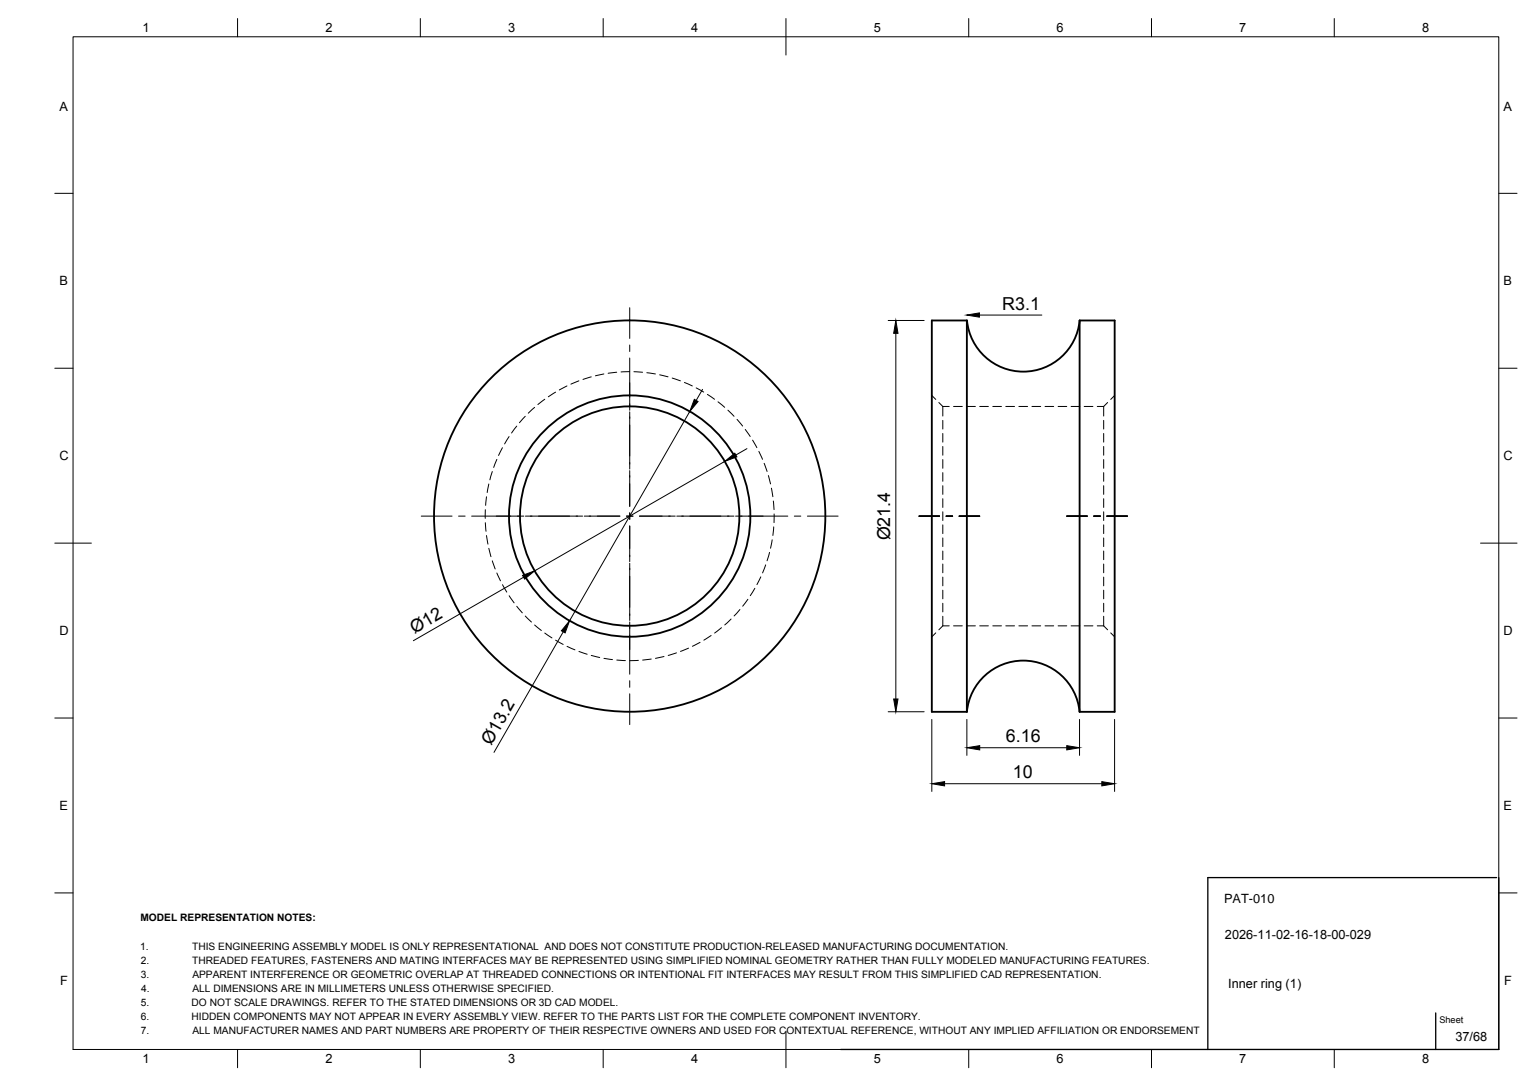
ISO-10303-21;
HEADER;
/* Generated by software containing ST-Developer
 * from STEP Tools, Inc. (www.steptools.com) 
 */

FILE_DESCRIPTION(
/* description */ ('Belt conveyor head drive unit'),
/* implementation_level */ '2;1');

FILE_NAME(
/* name */ 'Inner ring (1).step',
/* time_stamp */ '2026-10-28T03:26:19-07:00',
/* author */ (''),
/* organization */ (''),
/* preprocessor_version */ 'ST-DEVELOPER v20.2',
/* originating_system */ 'Autodesk Translation Framework v15.17.0.0',
/* authorisation */ '');

FILE_SCHEMA (('AUTOMOTIVE_DESIGN { 1 0 10303 214 3 1 1 }'));
ENDSEC;

DATA;
#10=MECHANICAL_DESIGN_GEOMETRIC_PRESENTATION_REPRESENTATION('',(#888),#27069);
#685=CONICAL_SURFACE('',#15366,0.63,0.785398163397448);
#686=CONICAL_SURFACE('',#15373,0.63,0.785398163397448);
#707=TOROIDAL_SURFACE('',#15355,1.1,0.309556);
#742=SHAPE_REPRESENTATION_RELATIONSHIP('SRR','None',#27388,#811);
#811=ADVANCED_BREP_SHAPE_REPRESENTATION('',(#972),#27030);
#888=STYLED_ITEM('',(#27797),#972);
#972=MANIFOLD_SOLID_BREP('Body1',#13754);
#1162=FACE_BOUND('',#2960,.T.);
#1163=FACE_BOUND('',#2963,.T.);
#1466=PLANE('',#15368);
#1467=PLANE('',#15371);
#2005=FACE_OUTER_BOUND('',#2955,.T.);
#2006=FACE_OUTER_BOUND('',#2956,.T.);
#2007=FACE_OUTER_BOUND('',#2957,.T.);
#2008=FACE_OUTER_BOUND('',#2958,.T.);
#2009=FACE_OUTER_BOUND('',#2959,.T.);
#2010=FACE_OUTER_BOUND('',#2961,.T.);
#2011=FACE_OUTER_BOUND('',#2962,.T.);
#2012=FACE_OUTER_BOUND('',#2964,.T.);
#2955=EDGE_LOOP('',(#10554,#10555,#10556,#10557,#10558,#10559));
#2956=EDGE_LOOP('',(#10560,#10561,#10562,#10563,#10564));
#2957=EDGE_LOOP('',(#10565,#10566,#10567,#10568));
#2958=EDGE_LOOP('',(#10569,#10570,#10571,#10572));
#2959=EDGE_LOOP('',(#10573));
#2960=EDGE_LOOP('',(#10574));
#2961=EDGE_LOOP('',(#10575,#10576,#10577,#10578,#10579));
#2962=EDGE_LOOP('',(#10580));
#2963=EDGE_LOOP('',(#10581));
#2964=EDGE_LOOP('',(#10582,#10583,#10584,#10585));
#3900=LINE('',#23073,#4692);
#3901=LINE('',#23079,#4693);
#3902=LINE('',#23083,#4694);
#3903=LINE('',#23089,#4695);
#3904=LINE('',#23094,#4696);
#4692=VECTOR('',#18436,1.070235);
#4693=VECTOR('',#18443,0.6);
#4694=VECTOR('',#18448,0.63);
#4695=VECTOR('',#18457,1.070235);
#4696=VECTOR('',#18464,0.63);
#5460=CIRCLE('',#15356,1.070235);
#5461=CIRCLE('',#15357,1.070235);
#5462=CIRCLE('',#15358,0.309556);
#5463=CIRCLE('',#15359,1.070235);
#5464=CIRCLE('',#15360,1.070235);
#5465=CIRCLE('',#15362,1.070235);
#5466=CIRCLE('',#15364,0.6);
#5467=CIRCLE('',#15365,0.6);
#5468=CIRCLE('',#15367,0.66);
#5469=CIRCLE('',#15370,1.070235);
#5470=CIRCLE('',#15372,0.66);
#6493=VERTEX_POINT('',#23062);
#6494=VERTEX_POINT('',#23063);
#6495=VERTEX_POINT('',#23066);
#6496=VERTEX_POINT('',#23068);
#6497=VERTEX_POINT('',#23072);
#6498=VERTEX_POINT('',#23076);
#6499=VERTEX_POINT('',#23078);
#6500=VERTEX_POINT('',#23082);
#6501=VERTEX_POINT('',#23087);
#6502=VERTEX_POINT('',#23091);
#7969=EDGE_CURVE('',#6493,#6494,#5460,.T.);
#7970=EDGE_CURVE('',#6494,#6493,#5461,.T.);
#7971=EDGE_CURVE('',#6494,#6495,#5462,.T.);
#7972=EDGE_CURVE('',#6496,#6495,#5463,.T.);
#7973=EDGE_CURVE('',#6495,#6496,#5464,.T.);
#7974=EDGE_CURVE('',#6496,#6497,#3900,.T.);
#7975=EDGE_CURVE('',#6497,#6497,#5465,.T.);
#7976=EDGE_CURVE('',#6498,#6498,#5466,.T.);
#7977=EDGE_CURVE('',#6498,#6499,#3901,.T.);
#7978=EDGE_CURVE('',#6499,#6499,#5467,.T.);
#7979=EDGE_CURVE('',#6499,#6500,#3902,.T.);
#7980=EDGE_CURVE('',#6500,#6500,#5468,.T.);
#7981=EDGE_CURVE('',#6501,#6501,#5469,.T.);
#7982=EDGE_CURVE('',#6501,#6493,#3903,.T.);
#7983=EDGE_CURVE('',#6502,#6502,#5470,.T.);
#7984=EDGE_CURVE('',#6502,#6498,#3904,.T.);
#10554=ORIENTED_EDGE('',*,*,#7969,.F.);
#10555=ORIENTED_EDGE('',*,*,#7970,.F.);
#10556=ORIENTED_EDGE('',*,*,#7971,.T.);
#10557=ORIENTED_EDGE('',*,*,#7972,.F.);
#10558=ORIENTED_EDGE('',*,*,#7973,.F.);
#10559=ORIENTED_EDGE('',*,*,#7971,.F.);
#10560=ORIENTED_EDGE('',*,*,#7972,.T.);
#10561=ORIENTED_EDGE('',*,*,#7973,.T.);
#10562=ORIENTED_EDGE('',*,*,#7974,.T.);
#10563=ORIENTED_EDGE('',*,*,#7975,.T.);
#10564=ORIENTED_EDGE('',*,*,#7974,.F.);
#10565=ORIENTED_EDGE('',*,*,#7976,.T.);
#10566=ORIENTED_EDGE('',*,*,#7977,.T.);
#10567=ORIENTED_EDGE('',*,*,#7978,.F.);
#10568=ORIENTED_EDGE('',*,*,#7977,.F.);
#10569=ORIENTED_EDGE('',*,*,#7978,.T.);
#10570=ORIENTED_EDGE('',*,*,#7979,.T.);
#10571=ORIENTED_EDGE('',*,*,#7980,.F.);
#10572=ORIENTED_EDGE('',*,*,#7979,.F.);
#10573=ORIENTED_EDGE('',*,*,#7975,.F.);
#10574=ORIENTED_EDGE('',*,*,#7980,.T.);
#10575=ORIENTED_EDGE('',*,*,#7981,.F.);
#10576=ORIENTED_EDGE('',*,*,#7982,.T.);
#10577=ORIENTED_EDGE('',*,*,#7969,.T.);
#10578=ORIENTED_EDGE('',*,*,#7970,.T.);
#10579=ORIENTED_EDGE('',*,*,#7982,.F.);
#10580=ORIENTED_EDGE('',*,*,#7981,.T.);
#10581=ORIENTED_EDGE('',*,*,#7983,.F.);
#10582=ORIENTED_EDGE('',*,*,#7983,.T.);
#10583=ORIENTED_EDGE('',*,*,#7984,.T.);
#10584=ORIENTED_EDGE('',*,*,#7976,.F.);
#10585=ORIENTED_EDGE('',*,*,#7984,.F.);
#12689=CYLINDRICAL_SURFACE('',#15361,1.070235);
#12690=CYLINDRICAL_SURFACE('',#15363,0.6);
#12691=CYLINDRICAL_SURFACE('',#15369,1.070235);
#13284=ADVANCED_FACE('',(#2005),#707,.F.);
#13285=ADVANCED_FACE('',(#2006),#12689,.T.);
#13286=ADVANCED_FACE('',(#2007),#12690,.F.);
#13287=ADVANCED_FACE('',(#2008),#685,.F.);
#13288=ADVANCED_FACE('',(#2009,#1162),#1466,.T.);
#13289=ADVANCED_FACE('',(#2010),#12691,.T.);
#13290=ADVANCED_FACE('',(#2011,#1163),#1467,.T.);
#13291=ADVANCED_FACE('',(#2012),#686,.F.);
#13754=CLOSED_SHELL('',(#13284,#13285,#13286,#13287,#13288,#13289,#13290,
#13291));
#15354=AXIS2_PLACEMENT_3D('',#23060,#18420,#18421);
#15355=AXIS2_PLACEMENT_3D('',#23061,#18422,#18423);
#15356=AXIS2_PLACEMENT_3D('',#23064,#18424,#18425);
#15357=AXIS2_PLACEMENT_3D('',#23065,#18426,#18427);
#15358=AXIS2_PLACEMENT_3D('',#23067,#18428,#18429);
#15359=AXIS2_PLACEMENT_3D('',#23069,#18430,#18431);
#15360=AXIS2_PLACEMENT_3D('',#23070,#18432,#18433);
#15361=AXIS2_PLACEMENT_3D('',#23071,#18434,#18435);
#15362=AXIS2_PLACEMENT_3D('',#23074,#18437,#18438);
#15363=AXIS2_PLACEMENT_3D('',#23075,#18439,#18440);
#15364=AXIS2_PLACEMENT_3D('',#23077,#18441,#18442);
#15365=AXIS2_PLACEMENT_3D('',#23080,#18444,#18445);
#15366=AXIS2_PLACEMENT_3D('',#23081,#18446,#18447);
#15367=AXIS2_PLACEMENT_3D('',#23084,#18449,#18450);
#15368=AXIS2_PLACEMENT_3D('',#23085,#18451,#18452);
#15369=AXIS2_PLACEMENT_3D('',#23086,#18453,#18454);
#15370=AXIS2_PLACEMENT_3D('',#23088,#18455,#18456);
#15371=AXIS2_PLACEMENT_3D('',#23090,#18458,#18459);
#15372=AXIS2_PLACEMENT_3D('',#23092,#18460,#18461);
#15373=AXIS2_PLACEMENT_3D('',#23093,#18462,#18463);
#18420=DIRECTION('axis',(0.,0.,1.));
#18421=DIRECTION('refdir',(1.,0.,0.));
#18422=DIRECTION('center_axis',(0.,-1.,0.));
#18423=DIRECTION('ref_axis',(0.,0.,-1.));
#18424=DIRECTION('center_axis',(0.,-1.,0.));
#18425=DIRECTION('ref_axis',(1.,0.,0.));
#18426=DIRECTION('center_axis',(0.,-1.,0.));
#18427=DIRECTION('ref_axis',(1.,0.,0.));
#18428=DIRECTION('center_axis',(1.,0.,1.22464679914735E-16));
#18429=DIRECTION('ref_axis',(-1.22464679914735E-16,0.,1.));
#18430=DIRECTION('center_axis',(0.,1.,0.));
#18431=DIRECTION('ref_axis',(1.,0.,0.));
#18432=DIRECTION('center_axis',(0.,1.,0.));
#18433=DIRECTION('ref_axis',(1.,0.,0.));
#18434=DIRECTION('center_axis',(0.,-1.,0.));
#18435=DIRECTION('ref_axis',(1.,0.,0.));
#18436=DIRECTION('',(0.,1.,0.));
#18437=DIRECTION('center_axis',(0.,-1.,0.));
#18438=DIRECTION('ref_axis',(1.,0.,0.));
#18439=DIRECTION('center_axis',(0.,-1.,0.));
#18440=DIRECTION('ref_axis',(1.,0.,0.));
#18441=DIRECTION('center_axis',(0.,-1.,0.));
#18442=DIRECTION('ref_axis',(1.,0.,0.));
#18443=DIRECTION('',(0.,1.,0.));
#18444=DIRECTION('center_axis',(0.,-1.,0.));
#18445=DIRECTION('ref_axis',(1.,0.,0.));
#18446=DIRECTION('center_axis',(0.,1.,0.));
#18447=DIRECTION('ref_axis',(1.,0.,0.));
#18448=DIRECTION('',(-0.707106781186548,0.707106781186547,-8.65956056235493E-17));
#18449=DIRECTION('center_axis',(0.,-1.,0.));
#18450=DIRECTION('ref_axis',(1.,0.,0.));
#18451=DIRECTION('center_axis',(0.,1.,0.));
#18452=DIRECTION('ref_axis',(0.,0.,1.));
#18453=DIRECTION('center_axis',(0.,-1.,0.));
#18454=DIRECTION('ref_axis',(1.,0.,0.));
#18455=DIRECTION('center_axis',(0.,-1.,0.));
#18456=DIRECTION('ref_axis',(1.,0.,0.));
#18457=DIRECTION('',(0.,1.,0.));
#18458=DIRECTION('center_axis',(0.,-1.,0.));
#18459=DIRECTION('ref_axis',(0.,0.,-1.));
#18460=DIRECTION('center_axis',(0.,-1.,0.));
#18461=DIRECTION('ref_axis',(1.,0.,0.));
#18462=DIRECTION('center_axis',(0.,-1.,0.));
#18463=DIRECTION('ref_axis',(1.,0.,0.));
#18464=DIRECTION('',(0.707106781186548,0.707106781186547,8.65956056235493E-17));
#23060=CARTESIAN_POINT('',(0.,0.,0.));
#23061=CARTESIAN_POINT('Origin',(0.,0.,0.));
#23062=CARTESIAN_POINT('',(-1.070235,-0.308121667383195,-1.31065986708547E-16));
#23063=CARTESIAN_POINT('',(-1.31065986708547E-16,-0.308121667383195,1.070235));
#23064=CARTESIAN_POINT('Origin',(0.,-0.308121667383195,0.));
#23065=CARTESIAN_POINT('Origin',(0.,-0.308121667383195,0.));
#23066=CARTESIAN_POINT('',(-1.31065986708547E-16,0.308121667383195,1.070235));
#23067=CARTESIAN_POINT('Origin',(-1.34711147906209E-16,0.,1.1));
#23068=CARTESIAN_POINT('',(-1.070235,0.308121667383195,1.31065986708547E-16));
#23069=CARTESIAN_POINT('Origin',(0.,0.308121667383195,0.));
#23070=CARTESIAN_POINT('Origin',(0.,0.308121667383195,0.));
#23071=CARTESIAN_POINT('Origin',(0.,0.,0.));
#23072=CARTESIAN_POINT('',(-1.070235,0.5,-1.31065986708547E-16));
#23073=CARTESIAN_POINT('',(-1.070235,0.,-1.31065986708547E-16));
#23074=CARTESIAN_POINT('Origin',(0.,0.5,0.));
#23075=CARTESIAN_POINT('Origin',(0.,0.,0.));
#23076=CARTESIAN_POINT('',(-0.6,-0.44,-7.34788079488412E-17));
#23077=CARTESIAN_POINT('Origin',(0.,-0.44,0.));
#23078=CARTESIAN_POINT('',(-0.6,0.44,-7.34788079488412E-17));
#23079=CARTESIAN_POINT('',(-0.6,0.,-7.34788079488412E-17));
#23080=CARTESIAN_POINT('Origin',(0.,0.44,0.));
#23081=CARTESIAN_POINT('Origin',(0.,0.47,0.));
#23082=CARTESIAN_POINT('',(-0.66,0.5,-8.08266887437253E-17));
#23083=CARTESIAN_POINT('',(-0.63,0.47,-7.71527483462832E-17));
#23084=CARTESIAN_POINT('Origin',(0.,0.5,0.));
#23085=CARTESIAN_POINT('Origin',(1.070235,0.5,0.));
#23086=CARTESIAN_POINT('Origin',(0.,0.,0.));
#23087=CARTESIAN_POINT('',(-1.070235,-0.5,-1.31065986708547E-16));
#23088=CARTESIAN_POINT('Origin',(0.,-0.5,0.));
#23089=CARTESIAN_POINT('',(-1.070235,0.,-1.31065986708547E-16));
#23090=CARTESIAN_POINT('Origin',(0.66,-0.5,0.));
#23091=CARTESIAN_POINT('',(-0.66,-0.5,-8.08266887437253E-17));
#23092=CARTESIAN_POINT('Origin',(0.,-0.5,0.));
#23093=CARTESIAN_POINT('Origin',(0.,-0.47,0.));
#23094=CARTESIAN_POINT('',(-0.63,-0.47,-7.71527483462832E-17));
#26953=UNCERTAINTY_MEASURE_WITH_UNIT(LENGTH_MEASURE(0.001),#27070,
'DISTANCE_ACCURACY_VALUE',
'Maximum model space distance between geometric entities at asserted c
onnectivities');
#26992=UNCERTAINTY_MEASURE_WITH_UNIT(LENGTH_MEASURE(0.001),#27070,
'DISTANCE_ACCURACY_VALUE',
'Maximum model space distance between geometric entities at asserted c
onnectivities');
#27030=(
GEOMETRIC_REPRESENTATION_CONTEXT(3)
GLOBAL_UNCERTAINTY_ASSIGNED_CONTEXT((#26953))
GLOBAL_UNIT_ASSIGNED_CONTEXT((#27070,#27072,#27073))
REPRESENTATION_CONTEXT('','3D')
);
#27069=(
GEOMETRIC_REPRESENTATION_CONTEXT(3)
GLOBAL_UNCERTAINTY_ASSIGNED_CONTEXT((#26992))
GLOBAL_UNIT_ASSIGNED_CONTEXT((#27070,#27072,#27073))
REPRESENTATION_CONTEXT('','3D')
);
#27070=(
LENGTH_UNIT()
NAMED_UNIT(*)
SI_UNIT(.CENTI.,.METRE.)
);
#27072=(
NAMED_UNIT(*)
PLANE_ANGLE_UNIT()
SI_UNIT($,.RADIAN.)
);
#27073=(
NAMED_UNIT(*)
SI_UNIT($,.STERADIAN.)
SOLID_ANGLE_UNIT()
);
#27111=SHAPE_DEFINITION_REPRESENTATION(#27192,#27388);
#27192=PRODUCT_DEFINITION_SHAPE('',$,#27465);
#27388=SHAPE_REPRESENTATION('',(#15354),#27030);
#27427=PRODUCT_DEFINITION_CONTEXT('part definition',#27657,'design');
#27465=PRODUCT_DEFINITION('Inner ring (1)','Inner ring (1)',#27541,#27427);
#27541=PRODUCT_DEFINITION_FORMATION('',$,#27696);
#27657=APPLICATION_CONTEXT(
'Core Data for Automotive Mechanical Design Process');
#27658=PRODUCT_CONTEXT('part definition',#27657,'mechanical');
#27696=PRODUCT('Inner ring (1)','Inner ring (1)','Inner ring (1)',(#27658));
#27791=COLOUR_RGB('Grey',0.48,0.52,0.57);
#27792=FILL_AREA_STYLE_COLOUR('',#27791);
#27793=FILL_AREA_STYLE('',(#27792));
#27794=SURFACE_STYLE_FILL_AREA(#27793);
#27795=SURFACE_SIDE_STYLE('',(#27794));
#27796=SURFACE_STYLE_USAGE(.BOTH.,#27795);
#27797=PRESENTATION_STYLE_ASSIGNMENT((#27796));
ENDSEC;
END-ISO-10303-21;
